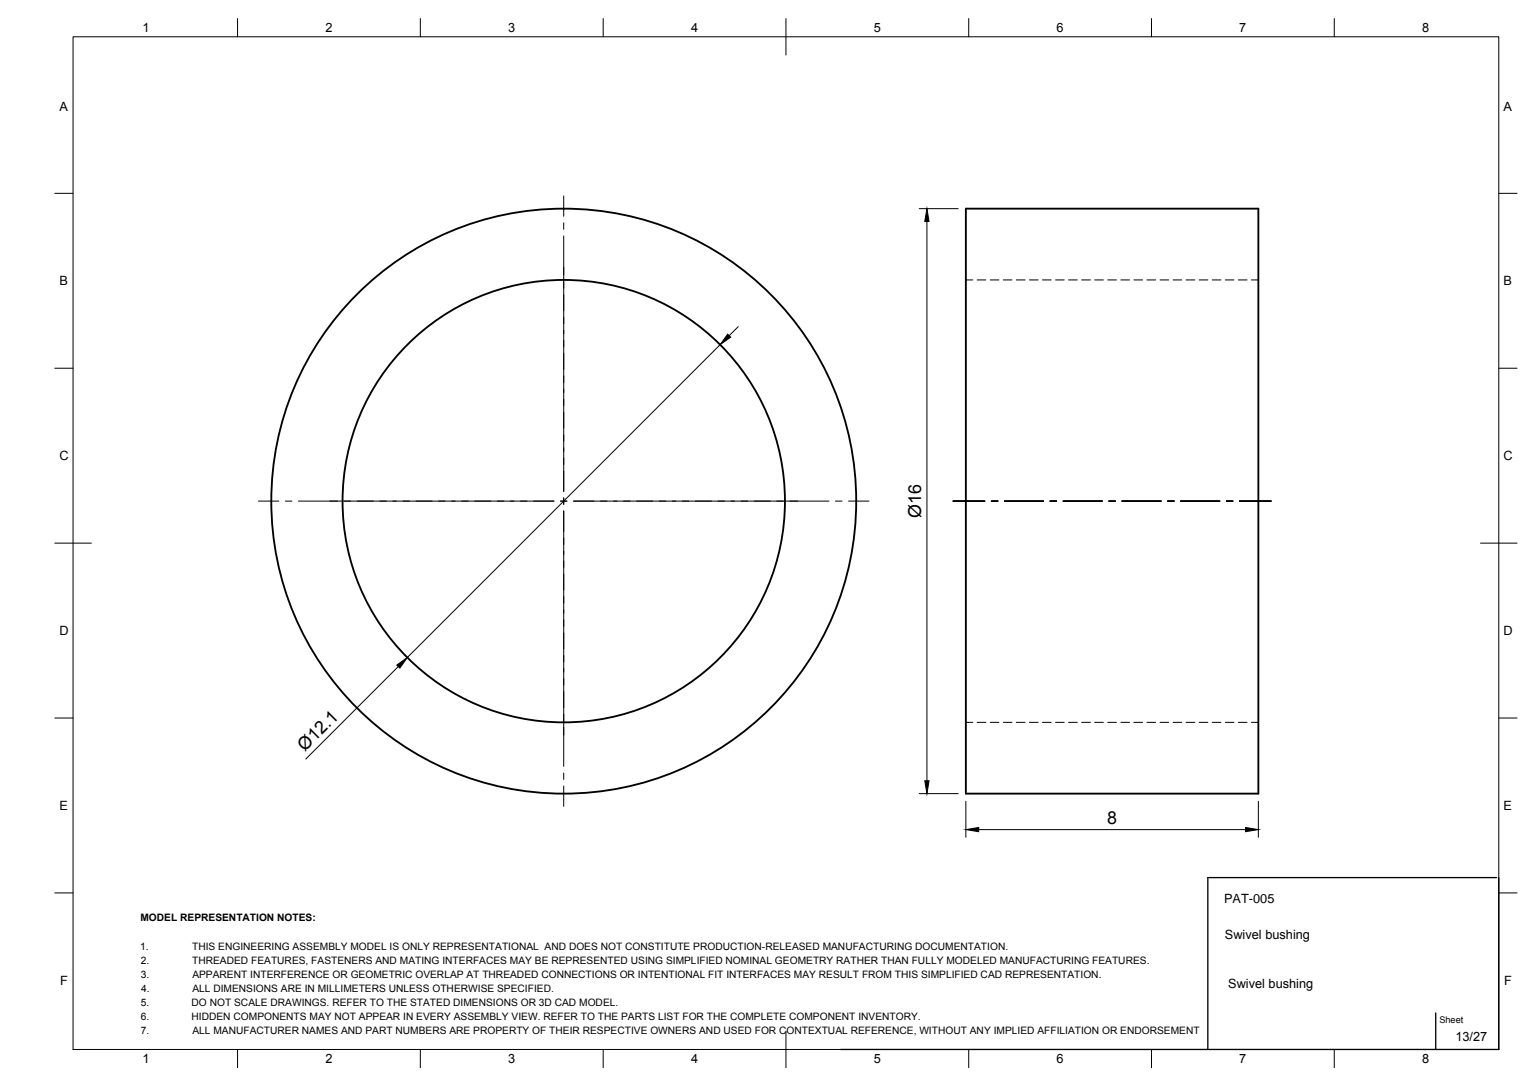
ISO-10303-21;
HEADER;
/* Generated by software containing ST-Developer
 * from STEP Tools, Inc. (www.steptools.com) 
 */

FILE_DESCRIPTION(
/* description */ ('Ball-race swivel caster'),
/* implementation_level */ '2;1');

FILE_NAME(
/* name */ 'Swivel bushing.step',
/* time_stamp */ '2026-10-29T16:15:51-07:00',
/* author */ (''),
/* organization */ (''),
/* preprocessor_version */ 'ST-DEVELOPER v20.2',
/* originating_system */ 'Autodesk Translation Framework v15.17.0.0',
/* authorisation */ '');

FILE_SCHEMA (('AUTOMOTIVE_DESIGN { 1 0 10303 214 3 1 1 }'));
ENDSEC;

DATA;
#10=MECHANICAL_DESIGN_GEOMETRIC_PRESENTATION_REPRESENTATION('',(#315),#7816);
#266=SHAPE_REPRESENTATION_RELATIONSHIP('SRR','None',#7913,#286);
#286=ADVANCED_BREP_SHAPE_REPRESENTATION('',(#351),#7802);
#315=STYLED_ITEM('',(#8090),#351);
#351=MANIFOLD_SOLID_BREP('Body1',#3721);
#414=FACE_BOUND('',#895,.T.);
#415=FACE_BOUND('',#897,.T.);
#481=PLANE('',#4261);
#482=PLANE('',#4262);
#638=FACE_OUTER_BOUND('',#892,.T.);
#639=FACE_OUTER_BOUND('',#893,.T.);
#640=FACE_OUTER_BOUND('',#894,.T.);
#641=FACE_OUTER_BOUND('',#896,.T.);
#892=EDGE_LOOP('',(#3079,#3080,#3081,#3082));
#893=EDGE_LOOP('',(#3083,#3084,#3085,#3086));
#894=EDGE_LOOP('',(#3087));
#895=EDGE_LOOP('',(#3088));
#896=EDGE_LOOP('',(#3089));
#897=EDGE_LOOP('',(#3090));
#1112=LINE('',#7048,#1267);
#1113=LINE('',#7054,#1268);
#1267=VECTOR('',#5180,0.605);
#1268=VECTOR('',#5187,0.8);
#1479=CIRCLE('',#4256,0.605);
#1480=CIRCLE('',#4257,0.605);
#1481=CIRCLE('',#4259,0.8);
#1482=CIRCLE('',#4260,0.8);
#1813=VERTEX_POINT('',#7045);
#1814=VERTEX_POINT('',#7047);
#1815=VERTEX_POINT('',#7051);
#1816=VERTEX_POINT('',#7053);
#2259=EDGE_CURVE('',#1813,#1813,#1479,.T.);
#2260=EDGE_CURVE('',#1813,#1814,#1112,.T.);
#2261=EDGE_CURVE('',#1814,#1814,#1480,.T.);
#2262=EDGE_CURVE('',#1815,#1815,#1481,.T.);
#2263=EDGE_CURVE('',#1815,#1816,#1113,.T.);
#2264=EDGE_CURVE('',#1816,#1816,#1482,.T.);
#3079=ORIENTED_EDGE('',*,*,#2259,.F.);
#3080=ORIENTED_EDGE('',*,*,#2260,.T.);
#3081=ORIENTED_EDGE('',*,*,#2261,.T.);
#3082=ORIENTED_EDGE('',*,*,#2260,.F.);
#3083=ORIENTED_EDGE('',*,*,#2262,.F.);
#3084=ORIENTED_EDGE('',*,*,#2263,.T.);
#3085=ORIENTED_EDGE('',*,*,#2264,.T.);
#3086=ORIENTED_EDGE('',*,*,#2263,.F.);
#3087=ORIENTED_EDGE('',*,*,#2262,.T.);
#3088=ORIENTED_EDGE('',*,*,#2259,.T.);
#3089=ORIENTED_EDGE('',*,*,#2264,.F.);
#3090=ORIENTED_EDGE('',*,*,#2261,.F.);
#3466=CYLINDRICAL_SURFACE('',#4255,0.605);
#3467=CYLINDRICAL_SURFACE('',#4258,0.8);
#3609=ADVANCED_FACE('',(#638),#3466,.F.);
#3610=ADVANCED_FACE('',(#639),#3467,.T.);
#3611=ADVANCED_FACE('',(#640,#414),#481,.T.);
#3612=ADVANCED_FACE('',(#641,#415),#482,.F.);
#3721=CLOSED_SHELL('',(#3609,#3610,#3611,#3612));
#4254=AXIS2_PLACEMENT_3D('',#7043,#5174,#5175);
#4255=AXIS2_PLACEMENT_3D('',#7044,#5176,#5177);
#4256=AXIS2_PLACEMENT_3D('',#7046,#5178,#5179);
#4257=AXIS2_PLACEMENT_3D('',#7049,#5181,#5182);
#4258=AXIS2_PLACEMENT_3D('',#7050,#5183,#5184);
#4259=AXIS2_PLACEMENT_3D('',#7052,#5185,#5186);
#4260=AXIS2_PLACEMENT_3D('',#7055,#5188,#5189);
#4261=AXIS2_PLACEMENT_3D('',#7056,#5190,#5191);
#4262=AXIS2_PLACEMENT_3D('',#7057,#5192,#5193);
#5174=DIRECTION('axis',(0.,0.,1.));
#5175=DIRECTION('refdir',(1.,0.,0.));
#5176=DIRECTION('center_axis',(0.,0.,1.));
#5177=DIRECTION('ref_axis',(1.,0.,0.));
#5178=DIRECTION('center_axis',(0.,0.,-1.));
#5179=DIRECTION('ref_axis',(1.,0.,0.));
#5180=DIRECTION('',(0.,0.,-1.));
#5181=DIRECTION('center_axis',(0.,0.,-1.));
#5182=DIRECTION('ref_axis',(1.,0.,0.));
#5183=DIRECTION('center_axis',(0.,0.,1.));
#5184=DIRECTION('ref_axis',(1.,0.,0.));
#5185=DIRECTION('center_axis',(0.,0.,1.));
#5186=DIRECTION('ref_axis',(1.,0.,0.));
#5187=DIRECTION('',(0.,0.,-1.));
#5188=DIRECTION('center_axis',(0.,0.,1.));
#5189=DIRECTION('ref_axis',(1.,0.,0.));
#5190=DIRECTION('center_axis',(0.,0.,1.));
#5191=DIRECTION('ref_axis',(1.,0.,0.));
#5192=DIRECTION('center_axis',(0.,0.,1.));
#5193=DIRECTION('ref_axis',(1.,0.,0.));
#7043=CARTESIAN_POINT('',(0.,0.,0.));
#7044=CARTESIAN_POINT('Origin',(-2.,0.,8.5));
#7045=CARTESIAN_POINT('',(-2.605,-7.40911313484149E-17,9.3));
#7046=CARTESIAN_POINT('Origin',(-2.,0.,9.3));
#7047=CARTESIAN_POINT('',(-2.605,-7.40911313484149E-17,8.5));
#7048=CARTESIAN_POINT('',(-2.605,-7.40911313484149E-17,8.5));
#7049=CARTESIAN_POINT('Origin',(-2.,0.,8.5));
#7050=CARTESIAN_POINT('Origin',(-2.,0.,8.5));
#7051=CARTESIAN_POINT('',(-2.8,-9.79717439317883E-17,9.3));
#7052=CARTESIAN_POINT('Origin',(-2.,0.,9.3));
#7053=CARTESIAN_POINT('',(-2.8,-9.79717439317883E-17,8.5));
#7054=CARTESIAN_POINT('',(-2.8,-9.79717439317883E-17,8.5));
#7055=CARTESIAN_POINT('Origin',(-2.,0.,8.5));
#7056=CARTESIAN_POINT('Origin',(-2.,0.,9.3));
#7057=CARTESIAN_POINT('Origin',(-2.,0.,8.5));
#7775=UNCERTAINTY_MEASURE_WITH_UNIT(LENGTH_MEASURE(0.001),#7817,
'DISTANCE_ACCURACY_VALUE',
'Maximum model space distance between geometric entities at asserted c
onnectivities');
#7789=UNCERTAINTY_MEASURE_WITH_UNIT(LENGTH_MEASURE(0.001),#7817,
'DISTANCE_ACCURACY_VALUE',
'Maximum model space distance between geometric entities at asserted c
onnectivities');
#7802=(
GEOMETRIC_REPRESENTATION_CONTEXT(3)
GLOBAL_UNCERTAINTY_ASSIGNED_CONTEXT((#7775))
GLOBAL_UNIT_ASSIGNED_CONTEXT((#7817,#7819,#7820))
REPRESENTATION_CONTEXT('','3D')
);
#7816=(
GEOMETRIC_REPRESENTATION_CONTEXT(3)
GLOBAL_UNCERTAINTY_ASSIGNED_CONTEXT((#7789))
GLOBAL_UNIT_ASSIGNED_CONTEXT((#7817,#7819,#7820))
REPRESENTATION_CONTEXT('','3D')
);
#7817=(
LENGTH_UNIT()
NAMED_UNIT(*)
SI_UNIT(.CENTI.,.METRE.)
);
#7819=(
NAMED_UNIT(*)
PLANE_ANGLE_UNIT()
SI_UNIT($,.RADIAN.)
);
#7820=(
NAMED_UNIT(*)
SI_UNIT($,.STERADIAN.)
SOLID_ANGLE_UNIT()
);
#7833=SHAPE_DEFINITION_REPRESENTATION(#7867,#7913);
#7867=PRODUCT_DEFINITION_SHAPE('',$,#7940);
#7913=SHAPE_REPRESENTATION('',(#4254),#7802);
#7927=PRODUCT_DEFINITION_CONTEXT('part definition',#8007,'design');
#7940=PRODUCT_DEFINITION('Swivel bushing','Swivel bushing',#7966,#7927);
#7966=PRODUCT_DEFINITION_FORMATION('',$,#8021);
#8007=APPLICATION_CONTEXT(
'Core Data for Automotive Mechanical Design Process');
#8008=PRODUCT_CONTEXT('part definition',#8007,'mechanical');
#8021=PRODUCT('Swivel bushing','Swivel bushing','Swivel bushing',(#8008));
#8084=COLOUR_RGB('Sky Blue',0.24,0.69,0.87);
#8085=FILL_AREA_STYLE_COLOUR('',#8084);
#8086=FILL_AREA_STYLE('',(#8085));
#8087=SURFACE_STYLE_FILL_AREA(#8086);
#8088=SURFACE_SIDE_STYLE('',(#8087));
#8089=SURFACE_STYLE_USAGE(.BOTH.,#8088);
#8090=PRESENTATION_STYLE_ASSIGNMENT((#8089));
ENDSEC;
END-ISO-10303-21;
